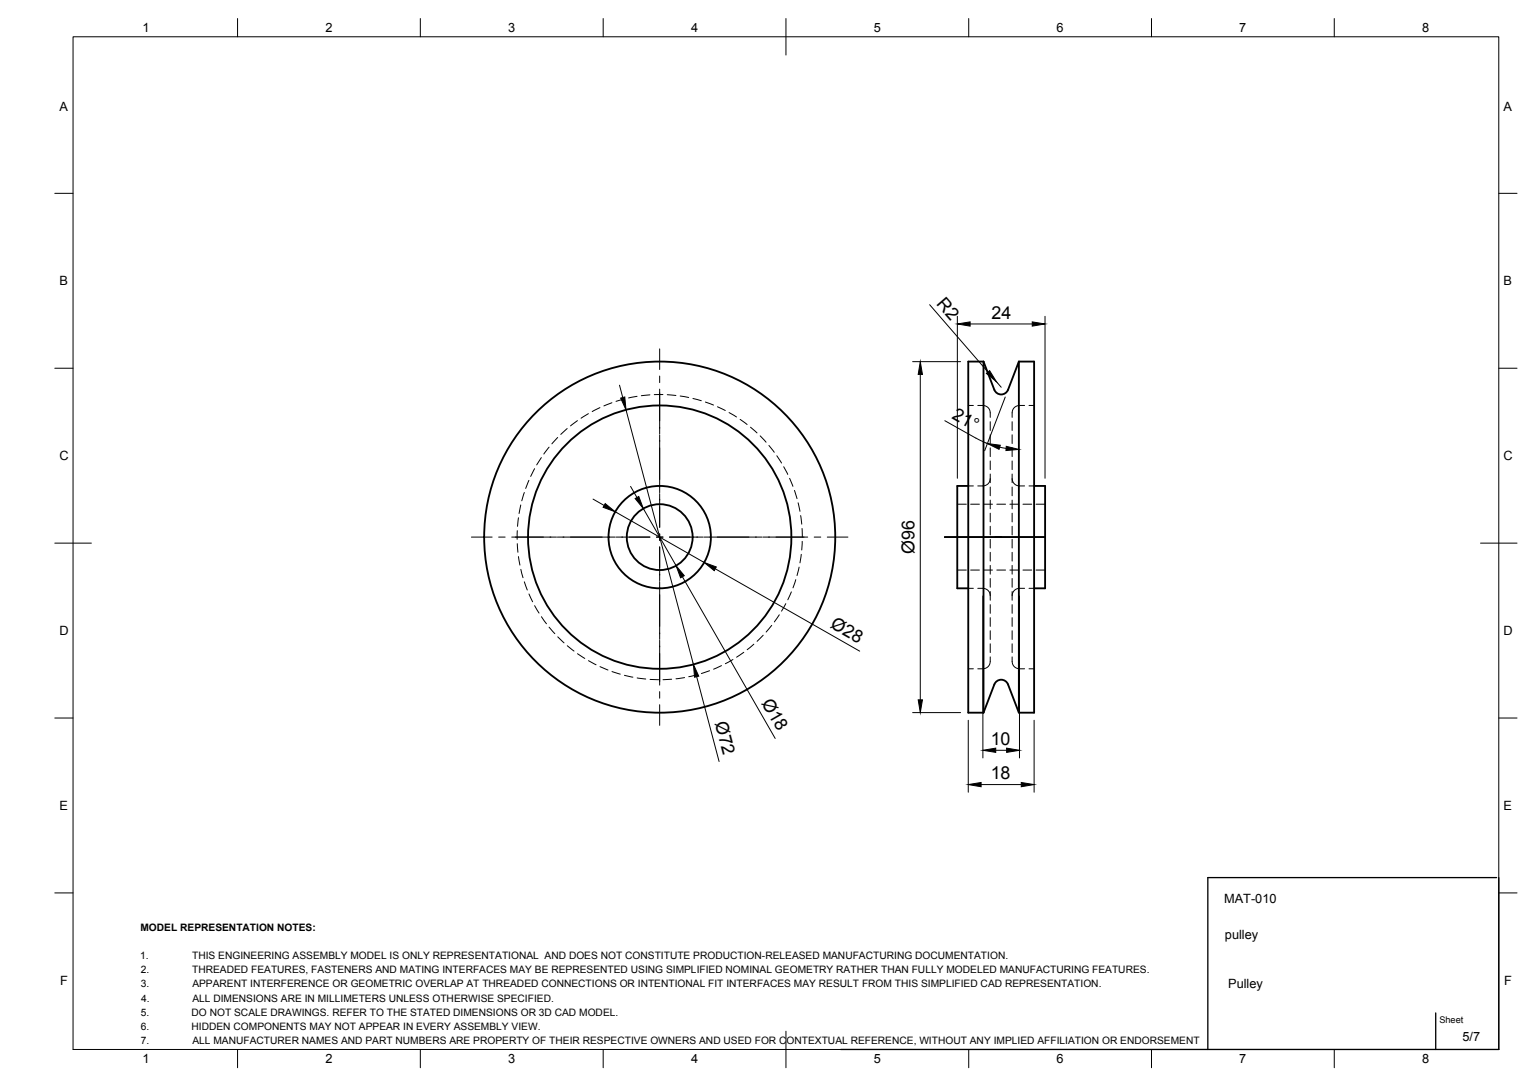
ISO-10303-21;
HEADER;
/* Generated by software containing ST-Developer
 * from STEP Tools, Inc. (www.steptools.com) 
 */

FILE_DESCRIPTION(
/* description */ ('STEP AP214'),
/* implementation_level */ '2;1');

FILE_NAME(
/* name */ 'Pulley.step',
/* time_stamp */ '2026-11-14T05:50:49-08:00',
/* author */ (''),
/* organization */ (''),
/* preprocessor_version */ 'ST-DEVELOPER v20.2',
/* originating_system */ 'Autodesk Translation Framework v15.17.0.0',
/* authorisation */ '');

FILE_SCHEMA (('AUTOMOTIVE_DESIGN { 1 0 10303 214 3 1 1 }'));
ENDSEC;

DATA;
#10=MECHANICAL_DESIGN_GEOMETRIC_PRESENTATION_REPRESENTATION('',(#159),#9903);
#129=CONICAL_SURFACE('',#2171,40.283264100914,1.20427718387609);
#130=CONICAL_SURFACE('',#2172,40.283264100914,1.20427718387609);
#136=TOROIDAL_SURFACE('',#2142,41.0000000000046,2.);
#137=TOROIDAL_SURFACE('',#2150,16.0000000000046,2.);
#138=TOROIDAL_SURFACE('',#2159,15.9999999999978,2.);
#139=TOROIDAL_SURFACE('',#2162,33.9999999999978,2.);
#140=TOROIDAL_SURFACE('',#2180,34.0000000000017,2.);
#145=SHAPE_REPRESENTATION_RELATIONSHIP('SRR','None',#9940,#152);
#152=ADVANCED_BREP_SHAPE_REPRESENTATION('',(#166),#9898);
#159=STYLED_ITEM('',(#9982),#166);
#166=MANIFOLD_SOLID_BREP('Body1',#2024);
#175=FACE_BOUND('',#404,.T.);
#176=FACE_BOUND('',#406,.T.);
#177=FACE_BOUND('',#408,.T.);
#178=FACE_BOUND('',#410,.T.);
#179=FACE_BOUND('',#412,.T.);
#180=FACE_BOUND('',#414,.T.);
#206=PLANE('',#2183);
#207=PLANE('',#2184);
#208=PLANE('',#2185);
#209=PLANE('',#2186);
#210=PLANE('',#2187);
#211=PLANE('',#2188);
#267=FACE_OUTER_BOUND('',#389,.T.);
#268=FACE_OUTER_BOUND('',#390,.T.);
#269=FACE_OUTER_BOUND('',#391,.T.);
#270=FACE_OUTER_BOUND('',#392,.T.);
#271=FACE_OUTER_BOUND('',#393,.T.);
#272=FACE_OUTER_BOUND('',#394,.T.);
#273=FACE_OUTER_BOUND('',#395,.T.);
#274=FACE_OUTER_BOUND('',#396,.T.);
#275=FACE_OUTER_BOUND('',#397,.T.);
#276=FACE_OUTER_BOUND('',#398,.T.);
#277=FACE_OUTER_BOUND('',#399,.T.);
#278=FACE_OUTER_BOUND('',#400,.T.);
#279=FACE_OUTER_BOUND('',#401,.T.);
#280=FACE_OUTER_BOUND('',#402,.T.);
#281=FACE_OUTER_BOUND('',#403,.T.);
#282=FACE_OUTER_BOUND('',#405,.T.);
#283=FACE_OUTER_BOUND('',#407,.T.);
#284=FACE_OUTER_BOUND('',#409,.T.);
#285=FACE_OUTER_BOUND('',#411,.T.);
#286=FACE_OUTER_BOUND('',#413,.T.);
#389=EDGE_LOOP('',(#1364,#1365,#1366,#1367,#1368));
#390=EDGE_LOOP('',(#1369,#1370,#1371,#1372));
#391=EDGE_LOOP('',(#1373,#1374,#1375,#1376));
#392=EDGE_LOOP('',(#1377,#1378,#1379,#1380));
#393=EDGE_LOOP('',(#1381,#1382,#1383,#1384));
#394=EDGE_LOOP('',(#1385,#1386,#1387,#1388));
#395=EDGE_LOOP('',(#1389,#1390,#1391,#1392));
#396=EDGE_LOOP('',(#1393,#1394,#1395,#1396));
#397=EDGE_LOOP('',(#1397,#1398,#1399,#1400));
#398=EDGE_LOOP('',(#1401,#1402,#1403,#1404));
#399=EDGE_LOOP('',(#1405,#1406,#1407,#1408,#1409,#1410));
#400=EDGE_LOOP('',(#1411,#1412,#1413,#1414,#1415));
#401=EDGE_LOOP('',(#1416,#1417,#1418,#1419));
#402=EDGE_LOOP('',(#1420,#1421,#1422,#1423));
#403=EDGE_LOOP('',(#1424));
#404=EDGE_LOOP('',(#1425));
#405=EDGE_LOOP('',(#1426));
#406=EDGE_LOOP('',(#1427));
#407=EDGE_LOOP('',(#1428));
#408=EDGE_LOOP('',(#1429));
#409=EDGE_LOOP('',(#1430));
#410=EDGE_LOOP('',(#1431));
#411=EDGE_LOOP('',(#1432));
#412=EDGE_LOOP('',(#1433));
#413=EDGE_LOOP('',(#1434));
#414=EDGE_LOOP('',(#1435));
#524=LINE('',#2952,#660);
#525=LINE('',#2962,#661);
#526=LINE('',#2968,#662);
#527=LINE('',#2982,#663);
#528=LINE('',#2988,#664);
#529=LINE('',#2991,#665);
#530=LINE('',#2996,#666);
#531=LINE('',#3000,#667);
#532=LINE('',#3006,#668);
#660=VECTOR('',#2413,9.);
#661=VECTOR('',#2426,14.0000000000046);
#662=VECTOR('',#2433,13.9999999999978);
#663=VECTOR('',#2452,35.9999999999978);
#664=VECTOR('',#2459,48.0000000000047);
#665=VECTOR('',#2464,40.283264100914);
#666=VECTOR('',#2469,40.283264100914);
#667=VECTOR('',#2474,48.0000000000047);
#668=VECTOR('',#2481,36.0000000000017);
#801=CIRCLE('',#2143,40.283264100914);
#802=CIRCLE('',#2144,2.);
#803=CIRCLE('',#2145,40.283264100914);
#804=CIRCLE('',#2146,40.283264100914);
#805=CIRCLE('',#2148,9.);
#806=CIRCLE('',#2149,9.);
#807=CIRCLE('',#2151,16.0000000000017);
#808=CIRCLE('',#2152,2.);
#809=CIRCLE('',#2153,14.0000000000046);
#810=CIRCLE('',#2155,14.0000000000046);
#811=CIRCLE('',#2157,13.9999999999978);
#812=CIRCLE('',#2158,13.9999999999978);
#813=CIRCLE('',#2160,2.);
#814=CIRCLE('',#2161,15.9999999999978);
#815=CIRCLE('',#2163,33.9999999999978);
#816=CIRCLE('',#2164,2.);
#817=CIRCLE('',#2165,35.9999999999978);
#818=CIRCLE('',#2167,35.9999999999978);
#819=CIRCLE('',#2169,48.0000000000047);
#820=CIRCLE('',#2170,48.0000000000047);
#821=CIRCLE('',#2173,48.0000000000047);
#822=CIRCLE('',#2174,48.0000000000047);
#823=CIRCLE('',#2176,48.0000000000047);
#824=CIRCLE('',#2178,36.0000000000017);
#825=CIRCLE('',#2179,36.0000000000017);
#826=CIRCLE('',#2181,2.);
#827=CIRCLE('',#2182,34.0000000000017);
#877=VERTEX_POINT('',#2941);
#878=VERTEX_POINT('',#2943);
#879=VERTEX_POINT('',#2945);
#880=VERTEX_POINT('',#2949);
#881=VERTEX_POINT('',#2951);
#882=VERTEX_POINT('',#2955);
#883=VERTEX_POINT('',#2957);
#884=VERTEX_POINT('',#2961);
#885=VERTEX_POINT('',#2965);
#886=VERTEX_POINT('',#2967);
#887=VERTEX_POINT('',#2971);
#888=VERTEX_POINT('',#2975);
#889=VERTEX_POINT('',#2977);
#890=VERTEX_POINT('',#2981);
#891=VERTEX_POINT('',#2985);
#892=VERTEX_POINT('',#2987);
#893=VERTEX_POINT('',#2993);
#894=VERTEX_POINT('',#2994);
#895=VERTEX_POINT('',#2999);
#896=VERTEX_POINT('',#3003);
#897=VERTEX_POINT('',#3005);
#898=VERTEX_POINT('',#3009);
#1063=EDGE_CURVE('',#877,#877,#801,.T.);
#1064=EDGE_CURVE('',#877,#878,#802,.T.);
#1065=EDGE_CURVE('',#878,#879,#803,.T.);
#1066=EDGE_CURVE('',#879,#878,#804,.T.);
#1067=EDGE_CURVE('',#880,#880,#805,.T.);
#1068=EDGE_CURVE('',#880,#881,#524,.T.);
#1069=EDGE_CURVE('',#881,#881,#806,.T.);
#1070=EDGE_CURVE('',#882,#882,#807,.T.);
#1071=EDGE_CURVE('',#882,#883,#808,.T.);
#1072=EDGE_CURVE('',#883,#883,#809,.T.);
#1073=EDGE_CURVE('',#883,#884,#525,.T.);
#1074=EDGE_CURVE('',#884,#884,#810,.T.);
#1075=EDGE_CURVE('',#885,#885,#811,.T.);
#1076=EDGE_CURVE('',#885,#886,#526,.T.);
#1077=EDGE_CURVE('',#886,#886,#812,.T.);
#1078=EDGE_CURVE('',#886,#887,#813,.T.);
#1079=EDGE_CURVE('',#887,#887,#814,.T.);
#1080=EDGE_CURVE('',#888,#888,#815,.T.);
#1081=EDGE_CURVE('',#888,#889,#816,.T.);
#1082=EDGE_CURVE('',#889,#889,#817,.T.);
#1083=EDGE_CURVE('',#889,#890,#527,.T.);
#1084=EDGE_CURVE('',#890,#890,#818,.T.);
#1085=EDGE_CURVE('',#891,#891,#819,.T.);
#1086=EDGE_CURVE('',#891,#892,#528,.T.);
#1087=EDGE_CURVE('',#892,#892,#820,.T.);
#1088=EDGE_CURVE('',#892,#877,#529,.T.);
#1089=EDGE_CURVE('',#893,#894,#821,.T.);
#1090=EDGE_CURVE('',#894,#879,#530,.T.);
#1091=EDGE_CURVE('',#894,#893,#822,.T.);
#1092=EDGE_CURVE('',#893,#895,#531,.T.);
#1093=EDGE_CURVE('',#895,#895,#823,.T.);
#1094=EDGE_CURVE('',#896,#896,#824,.T.);
#1095=EDGE_CURVE('',#896,#897,#532,.T.);
#1096=EDGE_CURVE('',#897,#897,#825,.T.);
#1097=EDGE_CURVE('',#897,#898,#826,.T.);
#1098=EDGE_CURVE('',#898,#898,#827,.T.);
#1364=ORIENTED_EDGE('',*,*,#1063,.F.);
#1365=ORIENTED_EDGE('',*,*,#1064,.T.);
#1366=ORIENTED_EDGE('',*,*,#1065,.T.);
#1367=ORIENTED_EDGE('',*,*,#1066,.T.);
#1368=ORIENTED_EDGE('',*,*,#1064,.F.);
#1369=ORIENTED_EDGE('',*,*,#1067,.T.);
#1370=ORIENTED_EDGE('',*,*,#1068,.T.);
#1371=ORIENTED_EDGE('',*,*,#1069,.T.);
#1372=ORIENTED_EDGE('',*,*,#1068,.F.);
#1373=ORIENTED_EDGE('',*,*,#1070,.F.);
#1374=ORIENTED_EDGE('',*,*,#1071,.T.);
#1375=ORIENTED_EDGE('',*,*,#1072,.T.);
#1376=ORIENTED_EDGE('',*,*,#1071,.F.);
#1377=ORIENTED_EDGE('',*,*,#1072,.F.);
#1378=ORIENTED_EDGE('',*,*,#1073,.T.);
#1379=ORIENTED_EDGE('',*,*,#1074,.T.);
#1380=ORIENTED_EDGE('',*,*,#1073,.F.);
#1381=ORIENTED_EDGE('',*,*,#1075,.F.);
#1382=ORIENTED_EDGE('',*,*,#1076,.T.);
#1383=ORIENTED_EDGE('',*,*,#1077,.T.);
#1384=ORIENTED_EDGE('',*,*,#1076,.F.);
#1385=ORIENTED_EDGE('',*,*,#1077,.F.);
#1386=ORIENTED_EDGE('',*,*,#1078,.T.);
#1387=ORIENTED_EDGE('',*,*,#1079,.T.);
#1388=ORIENTED_EDGE('',*,*,#1078,.F.);
#1389=ORIENTED_EDGE('',*,*,#1080,.F.);
#1390=ORIENTED_EDGE('',*,*,#1081,.T.);
#1391=ORIENTED_EDGE('',*,*,#1082,.T.);
#1392=ORIENTED_EDGE('',*,*,#1081,.F.);
#1393=ORIENTED_EDGE('',*,*,#1082,.F.);
#1394=ORIENTED_EDGE('',*,*,#1083,.T.);
#1395=ORIENTED_EDGE('',*,*,#1084,.T.);
#1396=ORIENTED_EDGE('',*,*,#1083,.F.);
#1397=ORIENTED_EDGE('',*,*,#1085,.F.);
#1398=ORIENTED_EDGE('',*,*,#1086,.T.);
#1399=ORIENTED_EDGE('',*,*,#1087,.T.);
#1400=ORIENTED_EDGE('',*,*,#1086,.F.);
#1401=ORIENTED_EDGE('',*,*,#1087,.F.);
#1402=ORIENTED_EDGE('',*,*,#1088,.T.);
#1403=ORIENTED_EDGE('',*,*,#1063,.T.);
#1404=ORIENTED_EDGE('',*,*,#1088,.F.);
#1405=ORIENTED_EDGE('',*,*,#1089,.T.);
#1406=ORIENTED_EDGE('',*,*,#1090,.T.);
#1407=ORIENTED_EDGE('',*,*,#1065,.F.);
#1408=ORIENTED_EDGE('',*,*,#1066,.F.);
#1409=ORIENTED_EDGE('',*,*,#1090,.F.);
#1410=ORIENTED_EDGE('',*,*,#1091,.T.);
#1411=ORIENTED_EDGE('',*,*,#1089,.F.);
#1412=ORIENTED_EDGE('',*,*,#1092,.T.);
#1413=ORIENTED_EDGE('',*,*,#1093,.T.);
#1414=ORIENTED_EDGE('',*,*,#1092,.F.);
#1415=ORIENTED_EDGE('',*,*,#1091,.F.);
#1416=ORIENTED_EDGE('',*,*,#1094,.F.);
#1417=ORIENTED_EDGE('',*,*,#1095,.T.);
#1418=ORIENTED_EDGE('',*,*,#1096,.T.);
#1419=ORIENTED_EDGE('',*,*,#1095,.F.);
#1420=ORIENTED_EDGE('',*,*,#1096,.F.);
#1421=ORIENTED_EDGE('',*,*,#1097,.T.);
#1422=ORIENTED_EDGE('',*,*,#1098,.T.);
#1423=ORIENTED_EDGE('',*,*,#1097,.F.);
#1424=ORIENTED_EDGE('',*,*,#1075,.T.);
#1425=ORIENTED_EDGE('',*,*,#1069,.F.);
#1426=ORIENTED_EDGE('',*,*,#1074,.F.);
#1427=ORIENTED_EDGE('',*,*,#1067,.F.);
#1428=ORIENTED_EDGE('',*,*,#1098,.F.);
#1429=ORIENTED_EDGE('',*,*,#1070,.T.);
#1430=ORIENTED_EDGE('',*,*,#1093,.F.);
#1431=ORIENTED_EDGE('',*,*,#1094,.T.);
#1432=ORIENTED_EDGE('',*,*,#1085,.T.);
#1433=ORIENTED_EDGE('',*,*,#1084,.F.);
#1434=ORIENTED_EDGE('',*,*,#1080,.T.);
#1435=ORIENTED_EDGE('',*,*,#1079,.F.);
#1861=CYLINDRICAL_SURFACE('',#2147,9.);
#1862=CYLINDRICAL_SURFACE('',#2154,14.0000000000046);
#1863=CYLINDRICAL_SURFACE('',#2156,13.9999999999978);
#1864=CYLINDRICAL_SURFACE('',#2166,35.9999999999978);
#1865=CYLINDRICAL_SURFACE('',#2168,48.0000000000047);
#1866=CYLINDRICAL_SURFACE('',#2175,48.0000000000047);
#1867=CYLINDRICAL_SURFACE('',#2177,36.0000000000017);
#1919=ADVANCED_FACE('',(#267),#136,.F.);
#1920=ADVANCED_FACE('',(#268),#1861,.F.);
#1921=ADVANCED_FACE('',(#269),#137,.F.);
#1922=ADVANCED_FACE('',(#270),#1862,.T.);
#1923=ADVANCED_FACE('',(#271),#1863,.T.);
#1924=ADVANCED_FACE('',(#272),#138,.F.);
#1925=ADVANCED_FACE('',(#273),#139,.F.);
#1926=ADVANCED_FACE('',(#274),#1864,.F.);
#1927=ADVANCED_FACE('',(#275),#1865,.T.);
#1928=ADVANCED_FACE('',(#276),#129,.T.);
#1929=ADVANCED_FACE('',(#277),#130,.T.);
#1930=ADVANCED_FACE('',(#278),#1866,.T.);
#1931=ADVANCED_FACE('',(#279),#1867,.F.);
#1932=ADVANCED_FACE('',(#280),#140,.F.);
#1933=ADVANCED_FACE('',(#281,#175),#206,.F.);
#1934=ADVANCED_FACE('',(#282,#176),#207,.F.);
#1935=ADVANCED_FACE('',(#283,#177),#208,.T.);
#1936=ADVANCED_FACE('',(#284,#178),#209,.T.);
#1937=ADVANCED_FACE('',(#285,#179),#210,.F.);
#1938=ADVANCED_FACE('',(#286,#180),#211,.F.);
#2024=CLOSED_SHELL('',(#1919,#1920,#1921,#1922,#1923,#1924,#1925,#1926,
#1927,#1928,#1929,#1930,#1931,#1932,#1933,#1934,#1935,#1936,#1937,#1938));
#2141=AXIS2_PLACEMENT_3D('',#2939,#2397,#2398);
#2142=AXIS2_PLACEMENT_3D('',#2940,#2399,#2400);
#2143=AXIS2_PLACEMENT_3D('',#2942,#2401,#2402);
#2144=AXIS2_PLACEMENT_3D('',#2944,#2403,#2404);
#2145=AXIS2_PLACEMENT_3D('',#2946,#2405,#2406);
#2146=AXIS2_PLACEMENT_3D('',#2947,#2407,#2408);
#2147=AXIS2_PLACEMENT_3D('',#2948,#2409,#2410);
#2148=AXIS2_PLACEMENT_3D('',#2950,#2411,#2412);
#2149=AXIS2_PLACEMENT_3D('',#2953,#2414,#2415);
#2150=AXIS2_PLACEMENT_3D('',#2954,#2416,#2417);
#2151=AXIS2_PLACEMENT_3D('',#2956,#2418,#2419);
#2152=AXIS2_PLACEMENT_3D('',#2958,#2420,#2421);
#2153=AXIS2_PLACEMENT_3D('',#2959,#2422,#2423);
#2154=AXIS2_PLACEMENT_3D('',#2960,#2424,#2425);
#2155=AXIS2_PLACEMENT_3D('',#2963,#2427,#2428);
#2156=AXIS2_PLACEMENT_3D('',#2964,#2429,#2430);
#2157=AXIS2_PLACEMENT_3D('',#2966,#2431,#2432);
#2158=AXIS2_PLACEMENT_3D('',#2969,#2434,#2435);
#2159=AXIS2_PLACEMENT_3D('',#2970,#2436,#2437);
#2160=AXIS2_PLACEMENT_3D('',#2972,#2438,#2439);
#2161=AXIS2_PLACEMENT_3D('',#2973,#2440,#2441);
#2162=AXIS2_PLACEMENT_3D('',#2974,#2442,#2443);
#2163=AXIS2_PLACEMENT_3D('',#2976,#2444,#2445);
#2164=AXIS2_PLACEMENT_3D('',#2978,#2446,#2447);
#2165=AXIS2_PLACEMENT_3D('',#2979,#2448,#2449);
#2166=AXIS2_PLACEMENT_3D('',#2980,#2450,#2451);
#2167=AXIS2_PLACEMENT_3D('',#2983,#2453,#2454);
#2168=AXIS2_PLACEMENT_3D('',#2984,#2455,#2456);
#2169=AXIS2_PLACEMENT_3D('',#2986,#2457,#2458);
#2170=AXIS2_PLACEMENT_3D('',#2989,#2460,#2461);
#2171=AXIS2_PLACEMENT_3D('',#2990,#2462,#2463);
#2172=AXIS2_PLACEMENT_3D('',#2992,#2465,#2466);
#2173=AXIS2_PLACEMENT_3D('',#2995,#2467,#2468);
#2174=AXIS2_PLACEMENT_3D('',#2997,#2470,#2471);
#2175=AXIS2_PLACEMENT_3D('',#2998,#2472,#2473);
#2176=AXIS2_PLACEMENT_3D('',#3001,#2475,#2476);
#2177=AXIS2_PLACEMENT_3D('',#3002,#2477,#2478);
#2178=AXIS2_PLACEMENT_3D('',#3004,#2479,#2480);
#2179=AXIS2_PLACEMENT_3D('',#3007,#2482,#2483);
#2180=AXIS2_PLACEMENT_3D('',#3008,#2484,#2485);
#2181=AXIS2_PLACEMENT_3D('',#3010,#2486,#2487);
#2182=AXIS2_PLACEMENT_3D('',#3011,#2488,#2489);
#2183=AXIS2_PLACEMENT_3D('',#3012,#2490,#2491);
#2184=AXIS2_PLACEMENT_3D('',#3013,#2492,#2493);
#2185=AXIS2_PLACEMENT_3D('',#3014,#2494,#2495);
#2186=AXIS2_PLACEMENT_3D('',#3015,#2496,#2497);
#2187=AXIS2_PLACEMENT_3D('',#3016,#2498,#2499);
#2188=AXIS2_PLACEMENT_3D('',#3017,#2500,#2501);
#2397=DIRECTION('axis',(0.,0.,1.));
#2398=DIRECTION('refdir',(1.,0.,0.));
#2399=DIRECTION('center_axis',(-1.,0.,0.));
#2400=DIRECTION('ref_axis',(0.,0.,1.));
#2401=DIRECTION('center_axis',(-1.,0.,0.));
#2402=DIRECTION('ref_axis',(0.,0.,1.));
#2403=DIRECTION('center_axis',(0.,1.,-1.22464679914735E-16));
#2404=DIRECTION('ref_axis',(0.,-1.22464679914735E-16,-1.));
#2405=DIRECTION('center_axis',(-1.,0.,0.));
#2406=DIRECTION('ref_axis',(0.,0.,1.));
#2407=DIRECTION('center_axis',(-1.,0.,0.));
#2408=DIRECTION('ref_axis',(0.,0.,1.));
#2409=DIRECTION('center_axis',(-1.,0.,0.));
#2410=DIRECTION('ref_axis',(0.,0.,1.));
#2411=DIRECTION('center_axis',(1.,0.,0.));
#2412=DIRECTION('ref_axis',(0.,0.,1.));
#2413=DIRECTION('',(-1.,0.,0.));
#2414=DIRECTION('center_axis',(-1.,0.,0.));
#2415=DIRECTION('ref_axis',(0.,0.,-1.));
#2416=DIRECTION('center_axis',(-1.,0.,0.));
#2417=DIRECTION('ref_axis',(0.,0.,1.));
#2418=DIRECTION('center_axis',(-1.,0.,0.));
#2419=DIRECTION('ref_axis',(0.,0.,1.));
#2420=DIRECTION('center_axis',(0.,1.,-1.22464679914735E-16));
#2421=DIRECTION('ref_axis',(0.,-1.22464679914735E-16,-1.));
#2422=DIRECTION('center_axis',(-1.,0.,0.));
#2423=DIRECTION('ref_axis',(0.,0.,1.));
#2424=DIRECTION('center_axis',(-1.,0.,0.));
#2425=DIRECTION('ref_axis',(0.,0.,1.));
#2426=DIRECTION('',(1.,0.,0.));
#2427=DIRECTION('center_axis',(-1.,0.,0.));
#2428=DIRECTION('ref_axis',(0.,0.,1.));
#2429=DIRECTION('center_axis',(-1.,0.,0.));
#2430=DIRECTION('ref_axis',(0.,0.,1.));
#2431=DIRECTION('center_axis',(-1.,0.,0.));
#2432=DIRECTION('ref_axis',(0.,0.,1.));
#2433=DIRECTION('',(1.,0.,0.));
#2434=DIRECTION('center_axis',(-1.,0.,0.));
#2435=DIRECTION('ref_axis',(0.,0.,1.));
#2436=DIRECTION('center_axis',(-1.,0.,0.));
#2437=DIRECTION('ref_axis',(0.,0.,1.));
#2438=DIRECTION('center_axis',(0.,1.,-1.22464679914735E-16));
#2439=DIRECTION('ref_axis',(0.,-1.22464679914735E-16,-1.));
#2440=DIRECTION('center_axis',(-1.,0.,0.));
#2441=DIRECTION('ref_axis',(0.,0.,1.));
#2442=DIRECTION('center_axis',(-1.,0.,0.));
#2443=DIRECTION('ref_axis',(0.,0.,1.));
#2444=DIRECTION('center_axis',(-1.,0.,0.));
#2445=DIRECTION('ref_axis',(0.,0.,1.));
#2446=DIRECTION('center_axis',(0.,1.,-1.22464679914735E-16));
#2447=DIRECTION('ref_axis',(0.,-1.22464679914735E-16,-1.));
#2448=DIRECTION('center_axis',(-1.,0.,0.));
#2449=DIRECTION('ref_axis',(0.,0.,1.));
#2450=DIRECTION('center_axis',(-1.,0.,0.));
#2451=DIRECTION('ref_axis',(0.,0.,1.));
#2452=DIRECTION('',(-1.,0.,0.));
#2453=DIRECTION('center_axis',(-1.,0.,0.));
#2454=DIRECTION('ref_axis',(0.,0.,1.));
#2455=DIRECTION('center_axis',(-1.,0.,0.));
#2456=DIRECTION('ref_axis',(0.,0.,1.));
#2457=DIRECTION('center_axis',(-1.,0.,0.));
#2458=DIRECTION('ref_axis',(0.,0.,1.));
#2459=DIRECTION('',(1.,0.,0.));
#2460=DIRECTION('center_axis',(-1.,0.,0.));
#2461=DIRECTION('ref_axis',(0.,0.,1.));
#2462=DIRECTION('center_axis',(-1.,0.,0.));
#2463=DIRECTION('ref_axis',(0.,0.,1.));
#2464=DIRECTION('',(0.358367949545298,1.14330628105642E-16,0.933580426497203));
#2465=DIRECTION('center_axis',(1.,0.,0.));
#2466=DIRECTION('ref_axis',(0.,0.,-1.));
#2467=DIRECTION('center_axis',(-1.,0.,0.));
#2468=DIRECTION('ref_axis',(0.,0.,1.));
#2469=DIRECTION('',(-0.358367949545298,1.14330628105642E-16,-0.933580426497203));
#2470=DIRECTION('center_axis',(-1.,0.,0.));
#2471=DIRECTION('ref_axis',(0.,0.,1.));
#2472=DIRECTION('center_axis',(-1.,0.,0.));
#2473=DIRECTION('ref_axis',(0.,0.,1.));
#2474=DIRECTION('',(1.,0.,0.));
#2475=DIRECTION('center_axis',(-1.,0.,0.));
#2476=DIRECTION('ref_axis',(0.,0.,1.));
#2477=DIRECTION('center_axis',(-1.,0.,0.));
#2478=DIRECTION('ref_axis',(0.,0.,1.));
#2479=DIRECTION('center_axis',(-1.,0.,0.));
#2480=DIRECTION('ref_axis',(0.,0.,1.));
#2481=DIRECTION('',(-1.,0.,0.));
#2482=DIRECTION('center_axis',(-1.,0.,0.));
#2483=DIRECTION('ref_axis',(0.,0.,1.));
#2484=DIRECTION('center_axis',(-1.,0.,0.));
#2485=DIRECTION('ref_axis',(0.,0.,1.));
#2486=DIRECTION('center_axis',(0.,1.,-1.22464679914735E-16));
#2487=DIRECTION('ref_axis',(0.,-1.22464679914735E-16,-1.));
#2488=DIRECTION('center_axis',(-1.,0.,0.));
#2489=DIRECTION('ref_axis',(0.,0.,1.));
#2490=DIRECTION('center_axis',(1.,0.,0.));
#2491=DIRECTION('ref_axis',(0.,0.,-1.));
#2492=DIRECTION('center_axis',(-1.,0.,0.));
#2493=DIRECTION('ref_axis',(0.,0.,1.));
#2494=DIRECTION('center_axis',(1.,0.,0.));
#2495=DIRECTION('ref_axis',(0.,0.,-1.));
#2496=DIRECTION('center_axis',(1.,0.,0.));
#2497=DIRECTION('ref_axis',(0.,0.,-1.));
#2498=DIRECTION('center_axis',(1.,0.,0.));
#2499=DIRECTION('ref_axis',(0.,0.,-1.));
#2500=DIRECTION('center_axis',(1.,0.,0.));
#2501=DIRECTION('ref_axis',(0.,0.,-1.));
#2939=CARTESIAN_POINT('',(0.,0.,0.));
#2940=CARTESIAN_POINT('Origin',(-2.4980018054066E-13,0.,0.));
#2941=CARTESIAN_POINT('',(-1.86716085299465,4.93327704403918E-15,-40.283264100914));
#2942=CARTESIAN_POINT('Origin',(-1.86716085299465,0.,0.));
#2943=CARTESIAN_POINT('',(1.86716085299415,-4.93327704403918E-15,-40.283264100914));
#2944=CARTESIAN_POINT('Origin',(-2.4980018054066E-13,-5.02105187650471E-15,
-41.0000000000046));
#2945=CARTESIAN_POINT('',(1.86716085299415,5.40579083997353E-15,40.283264100914));
#2946=CARTESIAN_POINT('Origin',(1.86716085299415,0.,0.));
#2947=CARTESIAN_POINT('Origin',(1.86716085299415,0.,0.));
#2948=CARTESIAN_POINT('Origin',(15.,0.,0.));
#2949=CARTESIAN_POINT('',(12.,-1.10218211923262E-15,-9.));
#2950=CARTESIAN_POINT('Origin',(12.,0.,0.));
#2951=CARTESIAN_POINT('',(-11.9999999999937,-1.10218211923262E-15,-9.));
#2952=CARTESIAN_POINT('',(15.,-1.10218211923262E-15,-9.));
#2953=CARTESIAN_POINT('Origin',(-11.9999999999937,0.,0.));
#2954=CARTESIAN_POINT('Origin',(5.0000000000226,0.,0.));
#2955=CARTESIAN_POINT('',(3.0000000000226,-1.95943487863597E-15,-16.0000000000017));
#2956=CARTESIAN_POINT('Origin',(3.0000000000226,0.,0.));
#2957=CARTESIAN_POINT('',(5.0000000000226,-1.71450551880685E-15,-14.0000000000046));
#2958=CARTESIAN_POINT('Origin',(5.0000000000226,-1.95943487863633E-15,-16.0000000000046));
#2959=CARTESIAN_POINT('Origin',(5.0000000000226,0.,0.));
#2960=CARTESIAN_POINT('Origin',(-11.9999999999937,0.,0.));
#2961=CARTESIAN_POINT('',(12.,-1.71450551880685E-15,-14.0000000000046));
#2962=CARTESIAN_POINT('',(-11.9999999999937,-1.71450551880685E-15,-14.0000000000046));
#2963=CARTESIAN_POINT('Origin',(12.,0.,0.));
#2964=CARTESIAN_POINT('Origin',(-11.9999999999937,0.,0.));
#2965=CARTESIAN_POINT('',(-11.9999999999937,-1.71450551880603E-15,-13.9999999999978));
#2966=CARTESIAN_POINT('Origin',(-11.9999999999937,0.,0.));
#2967=CARTESIAN_POINT('',(-4.99999999998797,-1.71450551880603E-15,-13.9999999999978));
#2968=CARTESIAN_POINT('',(-11.9999999999937,-1.71450551880603E-15,-13.9999999999978));
#2969=CARTESIAN_POINT('Origin',(-4.99999999998797,0.,0.));
#2970=CARTESIAN_POINT('Origin',(-4.99999999998797,0.,0.));
#2971=CARTESIAN_POINT('',(-2.99999999998797,-1.9594348786355E-15,-15.9999999999978));
#2972=CARTESIAN_POINT('Origin',(-4.99999999998797,-1.9594348786355E-15,
-15.9999999999978));
#2973=CARTESIAN_POINT('Origin',(-2.99999999998797,0.,0.));
#2974=CARTESIAN_POINT('Origin',(-4.99999999998797,0.,0.));
#2975=CARTESIAN_POINT('',(-2.99999999998797,-4.16379911710073E-15,-33.9999999999978));
#2976=CARTESIAN_POINT('Origin',(-2.99999999998797,0.,0.));
#2977=CARTESIAN_POINT('',(-4.99999999998797,-4.40872847693021E-15,-35.9999999999978));
#2978=CARTESIAN_POINT('Origin',(-4.99999999998797,-4.16379911710073E-15,
-33.9999999999978));
#2979=CARTESIAN_POINT('Origin',(-4.99999999998797,0.,0.));
#2980=CARTESIAN_POINT('Origin',(-11.9999999999937,0.,0.));
#2981=CARTESIAN_POINT('',(-8.99999999999736,-4.40872847693021E-15,-35.9999999999978));
#2982=CARTESIAN_POINT('',(-11.9999999999937,-4.40872847693021E-15,-35.9999999999978));
#2983=CARTESIAN_POINT('Origin',(-8.99999999999736,0.,0.));
#2984=CARTESIAN_POINT('Origin',(-11.9999999999937,0.,0.));
#2985=CARTESIAN_POINT('',(-8.99999999999736,-5.87830463590787E-15,-48.0000000000047));
#2986=CARTESIAN_POINT('Origin',(-8.99999999999736,0.,0.));
#2987=CARTESIAN_POINT('',(-4.82933823252224,-5.87830463590787E-15,-48.0000000000047));
#2988=CARTESIAN_POINT('',(-11.9999999999937,-5.87830463590787E-15,-48.0000000000047));
#2989=CARTESIAN_POINT('Origin',(-4.82933823252224,0.,0.));
#2990=CARTESIAN_POINT('Origin',(-1.86716085299465,0.,0.));
#2991=CARTESIAN_POINT('',(-1.86716085299465,-4.93327704403918E-15,-40.283264100914));
#2992=CARTESIAN_POINT('Origin',(1.86716085299415,0.,0.));
#2993=CARTESIAN_POINT('',(4.82933823252174,5.87830463590787E-15,-48.0000000000047));
#2994=CARTESIAN_POINT('',(4.82933823252174,-5.87830463590787E-15,48.0000000000047));
#2995=CARTESIAN_POINT('Origin',(4.82933823252174,0.,0.));
#2996=CARTESIAN_POINT('',(1.86716085299415,-4.93327704403918E-15,40.283264100914));
#2997=CARTESIAN_POINT('Origin',(4.82933823252174,0.,0.));
#2998=CARTESIAN_POINT('Origin',(-11.9999999999937,0.,0.));
#2999=CARTESIAN_POINT('',(9.00000000000556,-5.87830463590787E-15,-48.0000000000047));
#3000=CARTESIAN_POINT('',(-11.9999999999937,-5.87830463590787E-15,-48.0000000000047));
#3001=CARTESIAN_POINT('Origin',(9.00000000000556,0.,0.));
#3002=CARTESIAN_POINT('Origin',(-11.9999999999937,0.,0.));
#3003=CARTESIAN_POINT('',(9.00000000000556,-4.40872847693068E-15,-36.0000000000017));
#3004=CARTESIAN_POINT('Origin',(9.00000000000556,0.,0.));
#3005=CARTESIAN_POINT('',(5.0000000000226,-4.40872847693068E-15,-36.0000000000017));
#3006=CARTESIAN_POINT('',(-11.9999999999937,-4.40872847693068E-15,-36.0000000000017));
#3007=CARTESIAN_POINT('Origin',(5.0000000000226,0.,0.));
#3008=CARTESIAN_POINT('Origin',(5.0000000000226,0.,0.));
#3009=CARTESIAN_POINT('',(3.0000000000226,-4.16379911710121E-15,-34.0000000000017));
#3010=CARTESIAN_POINT('Origin',(5.0000000000226,-4.16379911710121E-15,-34.0000000000017));
#3011=CARTESIAN_POINT('Origin',(3.0000000000226,0.,0.));
#3012=CARTESIAN_POINT('Origin',(-11.9999999999937,0.,0.));
#3013=CARTESIAN_POINT('Origin',(12.,0.,0.));
#3014=CARTESIAN_POINT('Origin',(3.0000000000226,0.,0.));
#3015=CARTESIAN_POINT('Origin',(9.00000000000556,0.,0.));
#3016=CARTESIAN_POINT('Origin',(-8.99999999999736,0.,0.));
#3017=CARTESIAN_POINT('Origin',(-2.99999999998797,0.,0.));
#9889=UNCERTAINTY_MEASURE_WITH_UNIT(LENGTH_MEASURE(0.01),#9904,
'DISTANCE_ACCURACY_VALUE',
'Maximum model space distance between geometric entities at asserted c
onnectivities');
#9894=UNCERTAINTY_MEASURE_WITH_UNIT(LENGTH_MEASURE(0.01),#9904,
'DISTANCE_ACCURACY_VALUE',
'Maximum model space distance between geometric entities at asserted c
onnectivities');
#9898=(
GEOMETRIC_REPRESENTATION_CONTEXT(3)
GLOBAL_UNCERTAINTY_ASSIGNED_CONTEXT((#9889))
GLOBAL_UNIT_ASSIGNED_CONTEXT((#9904,#9906,#9907))
REPRESENTATION_CONTEXT('','3D')
);
#9903=(
GEOMETRIC_REPRESENTATION_CONTEXT(3)
GLOBAL_UNCERTAINTY_ASSIGNED_CONTEXT((#9894))
GLOBAL_UNIT_ASSIGNED_CONTEXT((#9904,#9906,#9907))
REPRESENTATION_CONTEXT('','3D')
);
#9904=(
LENGTH_UNIT()
NAMED_UNIT(*)
SI_UNIT(.MILLI.,.METRE.)
);
#9906=(
NAMED_UNIT(*)
PLANE_ANGLE_UNIT()
SI_UNIT($,.RADIAN.)
);
#9907=(
NAMED_UNIT(*)
SI_UNIT($,.STERADIAN.)
SOLID_ANGLE_UNIT()
);
#9911=SHAPE_DEFINITION_REPRESENTATION(#9919,#9940);
#9919=PRODUCT_DEFINITION_SHAPE('',$,#9949);
#9940=SHAPE_REPRESENTATION('',(#2141),#9898);
#9945=PRODUCT_DEFINITION_CONTEXT('part definition',#9971,'design');
#9949=PRODUCT_DEFINITION('pulley','Pulley',#9957,#9945);
#9957=PRODUCT_DEFINITION_FORMATION('',$,#9976);
#9971=APPLICATION_CONTEXT(
'Core Data for Automotive Mechanical Design Process');
#9972=PRODUCT_CONTEXT('part definition',#9971,'mechanical');
#9976=PRODUCT('pulley','Pulley',$,(#9972));
#9982=PRESENTATION_STYLE_ASSIGNMENT((#9987));
#9987=SURFACE_STYLE_USAGE(.BOTH.,#9992);
#9992=SURFACE_SIDE_STYLE('',(#9997));
#9997=SURFACE_STYLE_FILL_AREA(#10002);
#10002=FILL_AREA_STYLE('Opaque(97,158,199)',(#10007));
#10007=FILL_AREA_STYLE_COLOUR('Opaque(97,158,199)',#10012);
#10012=COLOUR_RGB('Opaque(97,158,199)',0.380392156862745,0.619607843137255,
0.780392156862745);
ENDSEC;
END-ISO-10303-21;
